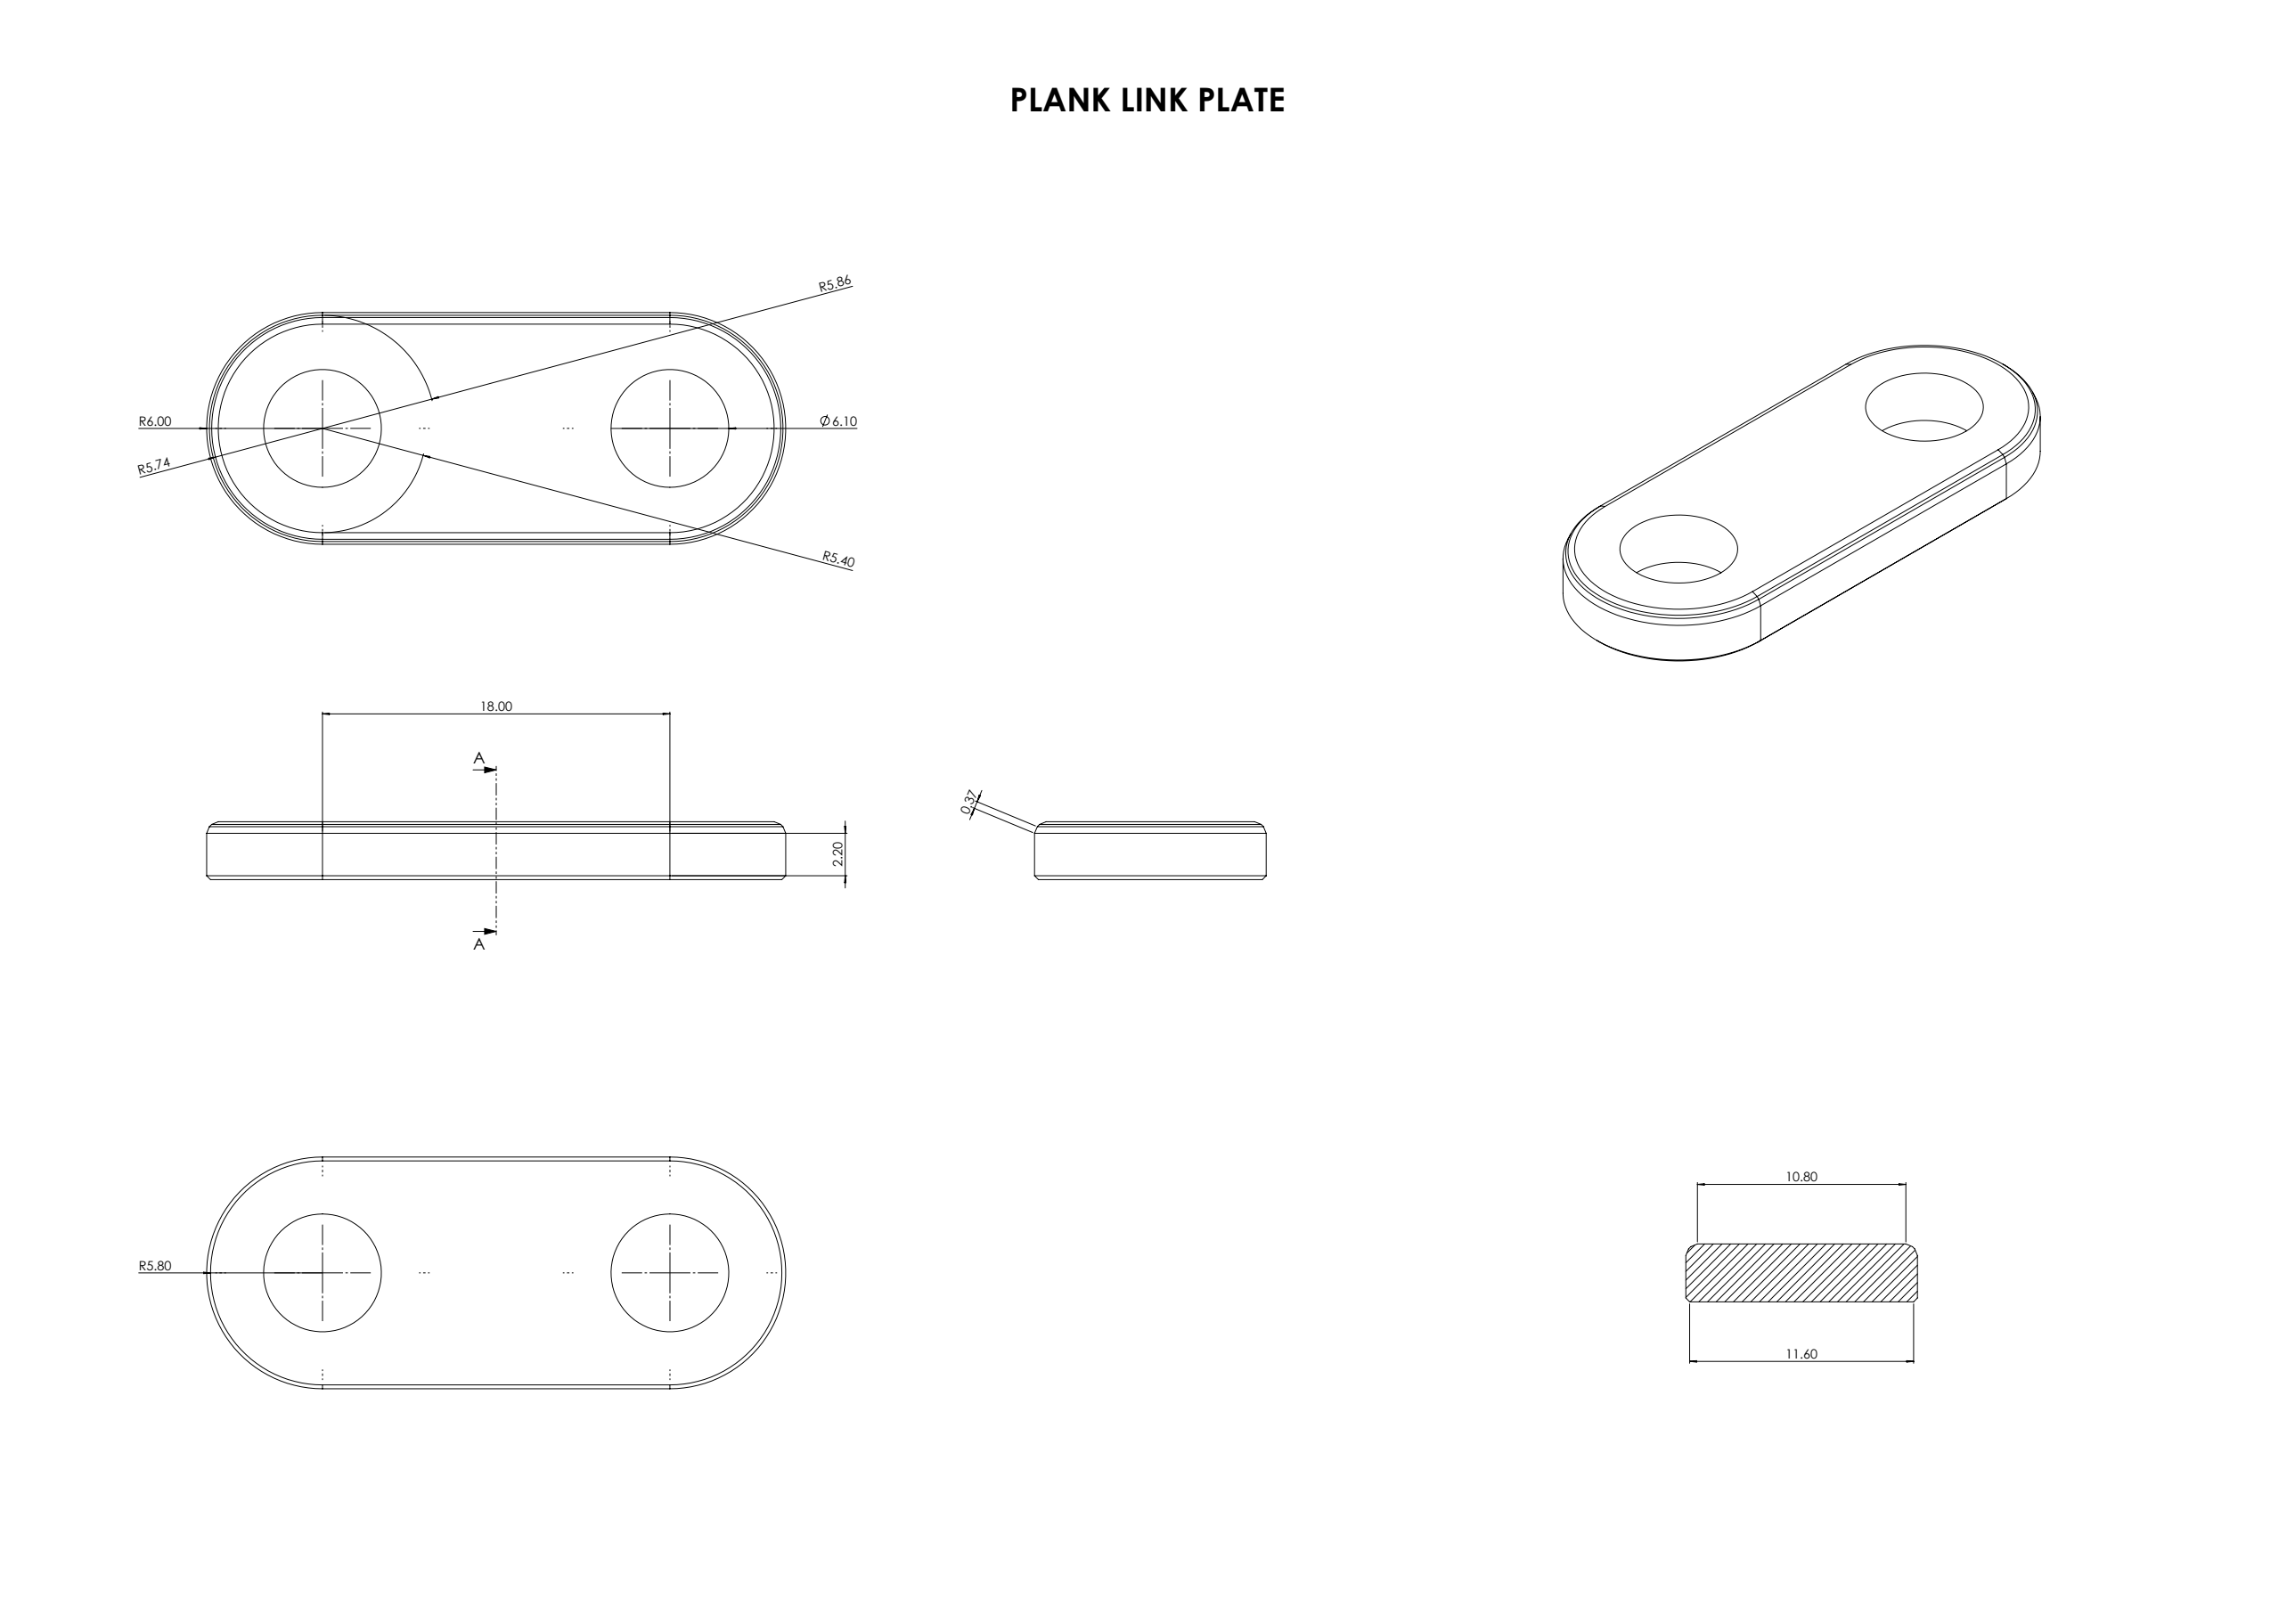
ISO-10303-21;
HEADER;
/* Generated by software containing ST-Developer
 * from STEP Tools, Inc. (www.steptools.com) 
 */

FILE_DESCRIPTION(
/* description */ (''),
/* implementation_level */ '2;1');

FILE_NAME(
/* name */ '09_Plank_Link_Plate.step',
/* time_stamp */ '2026-10-26T03:55:20-07:00',
/* author */ (''),
/* organization */ (''),
/* preprocessor_version */ 'ST-DEVELOPER v20.2',
/* originating_system */ 'Autodesk Translation Framework v15.15.0.0',
/* authorisation */ '');

FILE_SCHEMA (('AUTOMOTIVE_DESIGN { 1 0 10303 214 3 1 1 }'));
ENDSEC;

DATA;
#10=MECHANICAL_DESIGN_GEOMETRIC_PRESENTATION_REPRESENTATION('',(#191),#45236);
#151=SHAPE_REPRESENTATION_RELATIONSHIP('SRR','None',#45330,#171);
#171=ADVANCED_BREP_SHAPE_REPRESENTATION('',(#211),#45232);
#191=STYLED_ITEM('',(#45498),#211);
#211=MANIFOLD_SOLID_BREP('Body1',#16533);
#1051=FACE_BOUND('',#3821,.T.);
#1052=FACE_BOUND('',#3822,.T.);
#1053=FACE_BOUND('',#3835,.T.);
#1054=FACE_BOUND('',#3836,.T.);
#1529=PLANE('',#17991);
#1530=PLANE('',#17995);
#1531=PLANE('',#17996);
#1532=PLANE('',#17999);
#1533=PLANE('',#18002);
#1534=PLANE('',#18005);
#1535=PLANE('',#18011);
#1536=PLANE('',#18012);
#1537=PLANE('',#18015);
#1538=PLANE('',#18020);
#1539=PLANE('',#18023);
#1540=PLANE('',#18027);
#1801=CYLINDRICAL_SURFACE('',#17997,6.);
#1802=CYLINDRICAL_SURFACE('',#18024,3.05);
#1803=CYLINDRICAL_SURFACE('',#18025,3.05);
#1804=CYLINDRICAL_SURFACE('',#18026,6.);
#2728=FACE_OUTER_BOUND('',#3814,.T.);
#2729=FACE_OUTER_BOUND('',#3815,.T.);
#2730=FACE_OUTER_BOUND('',#3816,.T.);
#2731=FACE_OUTER_BOUND('',#3817,.T.);
#2732=FACE_OUTER_BOUND('',#3818,.T.);
#2733=FACE_OUTER_BOUND('',#3819,.T.);
#2734=FACE_OUTER_BOUND('',#3820,.T.);
#2735=FACE_OUTER_BOUND('',#3823,.T.);
#2736=FACE_OUTER_BOUND('',#3824,.T.);
#2737=FACE_OUTER_BOUND('',#3825,.T.);
#2738=FACE_OUTER_BOUND('',#3826,.T.);
#2739=FACE_OUTER_BOUND('',#3827,.T.);
#2740=FACE_OUTER_BOUND('',#3828,.T.);
#2741=FACE_OUTER_BOUND('',#3829,.T.);
#2742=FACE_OUTER_BOUND('',#3830,.T.);
#2743=FACE_OUTER_BOUND('',#3831,.T.);
#2744=FACE_OUTER_BOUND('',#3832,.T.);
#2745=FACE_OUTER_BOUND('',#3833,.T.);
#2746=FACE_OUTER_BOUND('',#3834,.T.);
#2747=FACE_OUTER_BOUND('',#3837,.T.);
#2748=FACE_OUTER_BOUND('',#3838,.T.);
#2749=FACE_OUTER_BOUND('',#3839,.T.);
#2750=FACE_OUTER_BOUND('',#3840,.T.);
#2751=FACE_OUTER_BOUND('',#3841,.T.);
#3814=EDGE_LOOP('',(#15244,#15245,#15246,#15247));
#3815=EDGE_LOOP('',(#15248,#15249,#15250,#15251));
#3816=EDGE_LOOP('',(#15252,#15253,#15254,#15255));
#3817=EDGE_LOOP('',(#15256,#15257,#15258,#15259));
#3818=EDGE_LOOP('',(#15260,#15261,#15262,#15263));
#3819=EDGE_LOOP('',(#15264,#15265,#15266,#15267));
#3820=EDGE_LOOP('',(#15268,#15269,#15270,#15271));
#3821=EDGE_LOOP('',(#15272));
#3822=EDGE_LOOP('',(#15273));
#3823=EDGE_LOOP('',(#15274,#15275,#15276,#15277));
#3824=EDGE_LOOP('',(#15278,#15279,#15280,#15281));
#3825=EDGE_LOOP('',(#15282,#15283,#15284,#15285));
#3826=EDGE_LOOP('',(#15286,#15287,#15288,#15289));
#3827=EDGE_LOOP('',(#15290,#15291,#15292,#15293));
#3828=EDGE_LOOP('',(#15294,#15295,#15296,#15297));
#3829=EDGE_LOOP('',(#15298,#15299,#15300,#15301));
#3830=EDGE_LOOP('',(#15302,#15303,#15304,#15305));
#3831=EDGE_LOOP('',(#15306,#15307,#15308,#15309));
#3832=EDGE_LOOP('',(#15310,#15311,#15312,#15313));
#3833=EDGE_LOOP('',(#15314,#15315,#15316,#15317));
#3834=EDGE_LOOP('',(#15318,#15319,#15320,#15321));
#3835=EDGE_LOOP('',(#15322));
#3836=EDGE_LOOP('',(#15323));
#3837=EDGE_LOOP('',(#15324,#15325,#15326,#15327));
#3838=EDGE_LOOP('',(#15328,#15329,#15330,#15331));
#3839=EDGE_LOOP('',(#15332,#15333,#15334,#15335));
#3840=EDGE_LOOP('',(#15336,#15337,#15338,#15339));
#3841=EDGE_LOOP('',(#15340,#15341,#15342,#15343));
#5125=LINE('',#44904,#6436);
#5126=LINE('',#44908,#6437);
#5127=LINE('',#44913,#6438);
#5128=LINE('',#44914,#6439);
#5129=LINE('',#44915,#6440);
#5130=LINE('',#44919,#6441);
#5131=LINE('',#44923,#6442);
#5132=LINE('',#44924,#6443);
#5133=LINE('',#44927,#6444);
#5134=LINE('',#44929,#6445);
#5135=LINE('',#44930,#6446);
#5136=LINE('',#44933,#6447);
#5137=LINE('',#44942,#6448);
#5138=LINE('',#44944,#6449);
#5139=LINE('',#44945,#6450);
#5140=LINE('',#44948,#6451);
#5141=LINE('',#44953,#6452);
#5142=LINE('',#44954,#6453);
#5143=LINE('',#44955,#6454);
#5144=LINE('',#44961,#6455);
#5145=LINE('',#44964,#6456);
#5146=LINE('',#44967,#6457);
#5147=LINE('',#44968,#6458);
#5148=LINE('',#44971,#6459);
#5149=LINE('',#44973,#6460);
#5150=LINE('',#44974,#6461);
#5151=LINE('',#44977,#6462);
#5152=LINE('',#44982,#6463);
#5153=LINE('',#44983,#6464);
#5154=LINE('',#44984,#6465);
#5155=LINE('',#44989,#6466);
#5156=LINE('',#44997,#6467);
#5157=LINE('',#44999,#6468);
#5158=LINE('',#45001,#6469);
#6436=VECTOR('',#21824,10.);
#6437=VECTOR('',#21827,10.);
#6438=VECTOR('',#21832,10.);
#6439=VECTOR('',#21833,10.);
#6440=VECTOR('',#21834,10.);
#6441=VECTOR('',#21837,10.);
#6442=VECTOR('',#21844,10.);
#6443=VECTOR('',#21845,10.);
#6444=VECTOR('',#21848,10.);
#6445=VECTOR('',#21849,10.);
#6446=VECTOR('',#21850,10.);
#6447=VECTOR('',#21853,10.);
#6448=VECTOR('',#21864,10.);
#6449=VECTOR('',#21865,10.);
#6450=VECTOR('',#21866,10.);
#6451=VECTOR('',#21869,10.);
#6452=VECTOR('',#21874,10.);
#6453=VECTOR('',#21875,10.);
#6454=VECTOR('',#21876,10.);
#6455=VECTOR('',#21885,10.);
#6456=VECTOR('',#21888,10.);
#6457=VECTOR('',#21891,10.);
#6458=VECTOR('',#21892,10.);
#6459=VECTOR('',#21895,10.);
#6460=VECTOR('',#21896,10.);
#6461=VECTOR('',#21897,10.);
#6462=VECTOR('',#21900,10.);
#6463=VECTOR('',#21905,10.);
#6464=VECTOR('',#21906,10.);
#6465=VECTOR('',#21907,10.);
#6466=VECTOR('',#21916,10.);
#6467=VECTOR('',#21927,3.05);
#6468=VECTOR('',#21930,3.05);
#6469=VECTOR('',#21933,10.);
#6922=CIRCLE('',#17989,6.);
#6923=CIRCLE('',#17990,5.8);
#6924=CIRCLE('',#17993,6.);
#6925=CIRCLE('',#17994,5.8);
#6926=CIRCLE('',#17998,6.);
#6927=CIRCLE('',#18000,3.05);
#6928=CIRCLE('',#18001,3.05);
#6929=CIRCLE('',#18004,5.85857864376269);
#6930=CIRCLE('',#18007,5.85857864376269);
#6931=CIRCLE('',#18008,6.);
#6932=CIRCLE('',#18010,5.74142135623731);
#6933=CIRCLE('',#18014,5.4);
#6934=CIRCLE('',#18017,5.74142135623731);
#6935=CIRCLE('',#18018,5.4);
#6936=CIRCLE('',#18021,3.05);
#6937=CIRCLE('',#18022,3.05);
#8395=VERTEX_POINT('',#44902);
#8396=VERTEX_POINT('',#44903);
#8397=VERTEX_POINT('',#44905);
#8398=VERTEX_POINT('',#44907);
#8399=VERTEX_POINT('',#44911);
#8400=VERTEX_POINT('',#44912);
#8401=VERTEX_POINT('',#44917);
#8402=VERTEX_POINT('',#44918);
#8403=VERTEX_POINT('',#44926);
#8404=VERTEX_POINT('',#44928);
#8405=VERTEX_POINT('',#44932);
#8406=VERTEX_POINT('',#44936);
#8407=VERTEX_POINT('',#44938);
#8408=VERTEX_POINT('',#44941);
#8409=VERTEX_POINT('',#44943);
#8410=VERTEX_POINT('',#44947);
#8411=VERTEX_POINT('',#44951);
#8412=VERTEX_POINT('',#44952);
#8413=VERTEX_POINT('',#44960);
#8414=VERTEX_POINT('',#44962);
#8415=VERTEX_POINT('',#44966);
#8416=VERTEX_POINT('',#44970);
#8417=VERTEX_POINT('',#44972);
#8418=VERTEX_POINT('',#44976);
#8419=VERTEX_POINT('',#44980);
#8420=VERTEX_POINT('',#44981);
#8421=VERTEX_POINT('',#44991);
#8422=VERTEX_POINT('',#44993);
#10685=EDGE_CURVE('',#8395,#8396,#5125,.T.);
#10686=EDGE_CURVE('',#8396,#8397,#6922,.T.);
#10687=EDGE_CURVE('',#8397,#8398,#5126,.T.);
#10688=EDGE_CURVE('',#8398,#8395,#6923,.T.);
#10689=EDGE_CURVE('',#8399,#8400,#5127,.T.);
#10690=EDGE_CURVE('',#8400,#8396,#5128,.T.);
#10691=EDGE_CURVE('',#8395,#8399,#5129,.T.);
#10692=EDGE_CURVE('',#8401,#8402,#5130,.T.);
#10693=EDGE_CURVE('',#8402,#8400,#6924,.T.);
#10694=EDGE_CURVE('',#8399,#8401,#6925,.T.);
#10695=EDGE_CURVE('',#8397,#8402,#5131,.T.);
#10696=EDGE_CURVE('',#8401,#8398,#5132,.T.);
#10697=EDGE_CURVE('',#8397,#8403,#5133,.T.);
#10698=EDGE_CURVE('',#8404,#8403,#5134,.T.);
#10699=EDGE_CURVE('',#8402,#8404,#5135,.T.);
#10700=EDGE_CURVE('',#8396,#8405,#5136,.T.);
#10701=EDGE_CURVE('',#8403,#8405,#6926,.T.);
#10702=EDGE_CURVE('',#8406,#8406,#6927,.T.);
#10703=EDGE_CURVE('',#8407,#8407,#6928,.T.);
#10704=EDGE_CURVE('',#8403,#8408,#5137,.T.);
#10705=EDGE_CURVE('',#8408,#8409,#5138,.T.);
#10706=EDGE_CURVE('',#8409,#8404,#5139,.T.);
#10707=EDGE_CURVE('',#8405,#8410,#5140,.T.);
#10708=EDGE_CURVE('',#8410,#8408,#6929,.T.);
#10709=EDGE_CURVE('',#8411,#8412,#5141,.T.);
#10710=EDGE_CURVE('',#8412,#8410,#5142,.T.);
#10711=EDGE_CURVE('',#8405,#8411,#5143,.T.);
#10712=EDGE_CURVE('',#8409,#8412,#6930,.T.);
#10713=EDGE_CURVE('',#8411,#8404,#6931,.T.);
#10714=EDGE_CURVE('',#8413,#8409,#5144,.T.);
#10715=EDGE_CURVE('',#8414,#8413,#6932,.T.);
#10716=EDGE_CURVE('',#8412,#8414,#5145,.T.);
#10717=EDGE_CURVE('',#8408,#8415,#5146,.T.);
#10718=EDGE_CURVE('',#8413,#8415,#5147,.T.);
#10719=EDGE_CURVE('',#8416,#8413,#5148,.T.);
#10720=EDGE_CURVE('',#8415,#8417,#5149,.T.);
#10721=EDGE_CURVE('',#8417,#8416,#5150,.T.);
#10722=EDGE_CURVE('',#8418,#8414,#5151,.T.);
#10723=EDGE_CURVE('',#8416,#8418,#6933,.T.);
#10724=EDGE_CURVE('',#8419,#8420,#5152,.T.);
#10725=EDGE_CURVE('',#8420,#8414,#5153,.T.);
#10726=EDGE_CURVE('',#8418,#8419,#5154,.T.);
#10727=EDGE_CURVE('',#8415,#8420,#6934,.T.);
#10728=EDGE_CURVE('',#8419,#8417,#6935,.T.);
#10729=EDGE_CURVE('',#8410,#8420,#5155,.T.);
#10730=EDGE_CURVE('',#8421,#8421,#6936,.T.);
#10731=EDGE_CURVE('',#8422,#8422,#6937,.T.);
#10732=EDGE_CURVE('',#8407,#8421,#5156,.T.);
#10733=EDGE_CURVE('',#8406,#8422,#5157,.T.);
#10734=EDGE_CURVE('',#8400,#8411,#5158,.T.);
#15244=ORIENTED_EDGE('',*,*,#10685,.T.);
#15245=ORIENTED_EDGE('',*,*,#10686,.T.);
#15246=ORIENTED_EDGE('',*,*,#10687,.T.);
#15247=ORIENTED_EDGE('',*,*,#10688,.T.);
#15248=ORIENTED_EDGE('',*,*,#10689,.T.);
#15249=ORIENTED_EDGE('',*,*,#10690,.T.);
#15250=ORIENTED_EDGE('',*,*,#10685,.F.);
#15251=ORIENTED_EDGE('',*,*,#10691,.T.);
#15252=ORIENTED_EDGE('',*,*,#10692,.T.);
#15253=ORIENTED_EDGE('',*,*,#10693,.T.);
#15254=ORIENTED_EDGE('',*,*,#10689,.F.);
#15255=ORIENTED_EDGE('',*,*,#10694,.T.);
#15256=ORIENTED_EDGE('',*,*,#10687,.F.);
#15257=ORIENTED_EDGE('',*,*,#10695,.T.);
#15258=ORIENTED_EDGE('',*,*,#10692,.F.);
#15259=ORIENTED_EDGE('',*,*,#10696,.T.);
#15260=ORIENTED_EDGE('',*,*,#10695,.F.);
#15261=ORIENTED_EDGE('',*,*,#10697,.T.);
#15262=ORIENTED_EDGE('',*,*,#10698,.F.);
#15263=ORIENTED_EDGE('',*,*,#10699,.F.);
#15264=ORIENTED_EDGE('',*,*,#10686,.F.);
#15265=ORIENTED_EDGE('',*,*,#10700,.T.);
#15266=ORIENTED_EDGE('',*,*,#10701,.F.);
#15267=ORIENTED_EDGE('',*,*,#10697,.F.);
#15268=ORIENTED_EDGE('',*,*,#10688,.F.);
#15269=ORIENTED_EDGE('',*,*,#10696,.F.);
#15270=ORIENTED_EDGE('',*,*,#10694,.F.);
#15271=ORIENTED_EDGE('',*,*,#10691,.F.);
#15272=ORIENTED_EDGE('',*,*,#10702,.T.);
#15273=ORIENTED_EDGE('',*,*,#10703,.T.);
#15274=ORIENTED_EDGE('',*,*,#10704,.T.);
#15275=ORIENTED_EDGE('',*,*,#10705,.T.);
#15276=ORIENTED_EDGE('',*,*,#10706,.T.);
#15277=ORIENTED_EDGE('',*,*,#10698,.T.);
#15278=ORIENTED_EDGE('',*,*,#10707,.T.);
#15279=ORIENTED_EDGE('',*,*,#10708,.T.);
#15280=ORIENTED_EDGE('',*,*,#10704,.F.);
#15281=ORIENTED_EDGE('',*,*,#10701,.T.);
#15282=ORIENTED_EDGE('',*,*,#10709,.T.);
#15283=ORIENTED_EDGE('',*,*,#10710,.T.);
#15284=ORIENTED_EDGE('',*,*,#10707,.F.);
#15285=ORIENTED_EDGE('',*,*,#10711,.T.);
#15286=ORIENTED_EDGE('',*,*,#10706,.F.);
#15287=ORIENTED_EDGE('',*,*,#10712,.T.);
#15288=ORIENTED_EDGE('',*,*,#10709,.F.);
#15289=ORIENTED_EDGE('',*,*,#10713,.T.);
#15290=ORIENTED_EDGE('',*,*,#10712,.F.);
#15291=ORIENTED_EDGE('',*,*,#10714,.F.);
#15292=ORIENTED_EDGE('',*,*,#10715,.F.);
#15293=ORIENTED_EDGE('',*,*,#10716,.F.);
#15294=ORIENTED_EDGE('',*,*,#10705,.F.);
#15295=ORIENTED_EDGE('',*,*,#10717,.T.);
#15296=ORIENTED_EDGE('',*,*,#10718,.F.);
#15297=ORIENTED_EDGE('',*,*,#10714,.T.);
#15298=ORIENTED_EDGE('',*,*,#10719,.T.);
#15299=ORIENTED_EDGE('',*,*,#10718,.T.);
#15300=ORIENTED_EDGE('',*,*,#10720,.T.);
#15301=ORIENTED_EDGE('',*,*,#10721,.T.);
#15302=ORIENTED_EDGE('',*,*,#10722,.T.);
#15303=ORIENTED_EDGE('',*,*,#10715,.T.);
#15304=ORIENTED_EDGE('',*,*,#10719,.F.);
#15305=ORIENTED_EDGE('',*,*,#10723,.T.);
#15306=ORIENTED_EDGE('',*,*,#10724,.T.);
#15307=ORIENTED_EDGE('',*,*,#10725,.T.);
#15308=ORIENTED_EDGE('',*,*,#10722,.F.);
#15309=ORIENTED_EDGE('',*,*,#10726,.T.);
#15310=ORIENTED_EDGE('',*,*,#10720,.F.);
#15311=ORIENTED_EDGE('',*,*,#10727,.T.);
#15312=ORIENTED_EDGE('',*,*,#10724,.F.);
#15313=ORIENTED_EDGE('',*,*,#10728,.T.);
#15314=ORIENTED_EDGE('',*,*,#10708,.F.);
#15315=ORIENTED_EDGE('',*,*,#10729,.T.);
#15316=ORIENTED_EDGE('',*,*,#10727,.F.);
#15317=ORIENTED_EDGE('',*,*,#10717,.F.);
#15318=ORIENTED_EDGE('',*,*,#10721,.F.);
#15319=ORIENTED_EDGE('',*,*,#10728,.F.);
#15320=ORIENTED_EDGE('',*,*,#10726,.F.);
#15321=ORIENTED_EDGE('',*,*,#10723,.F.);
#15322=ORIENTED_EDGE('',*,*,#10730,.T.);
#15323=ORIENTED_EDGE('',*,*,#10731,.T.);
#15324=ORIENTED_EDGE('',*,*,#10710,.F.);
#15325=ORIENTED_EDGE('',*,*,#10716,.T.);
#15326=ORIENTED_EDGE('',*,*,#10725,.F.);
#15327=ORIENTED_EDGE('',*,*,#10729,.F.);
#15328=ORIENTED_EDGE('',*,*,#10703,.F.);
#15329=ORIENTED_EDGE('',*,*,#10732,.T.);
#15330=ORIENTED_EDGE('',*,*,#10730,.F.);
#15331=ORIENTED_EDGE('',*,*,#10732,.F.);
#15332=ORIENTED_EDGE('',*,*,#10702,.F.);
#15333=ORIENTED_EDGE('',*,*,#10733,.T.);
#15334=ORIENTED_EDGE('',*,*,#10731,.F.);
#15335=ORIENTED_EDGE('',*,*,#10733,.F.);
#15336=ORIENTED_EDGE('',*,*,#10693,.F.);
#15337=ORIENTED_EDGE('',*,*,#10699,.T.);
#15338=ORIENTED_EDGE('',*,*,#10713,.F.);
#15339=ORIENTED_EDGE('',*,*,#10734,.F.);
#15340=ORIENTED_EDGE('',*,*,#10690,.F.);
#15341=ORIENTED_EDGE('',*,*,#10734,.T.);
#15342=ORIENTED_EDGE('',*,*,#10711,.F.);
#15343=ORIENTED_EDGE('',*,*,#10700,.F.);
#15530=CONICAL_SURFACE('',#17988,5.9,0.785398163397448);
#15531=CONICAL_SURFACE('',#17992,5.9,0.785398163397448);
#15532=CONICAL_SURFACE('',#18003,5.92928932188135,0.392699081698723);
#15533=CONICAL_SURFACE('',#18006,5.92928932188134,0.392699081698725);
#15534=CONICAL_SURFACE('',#18009,5.8,0.785398163397448);
#15535=CONICAL_SURFACE('',#18013,5.57071067811865,1.17809724509617);
#15536=CONICAL_SURFACE('',#18016,5.57071067811865,1.17809724509617);
#15537=CONICAL_SURFACE('',#18019,5.8,0.785398163397448);
#16456=ADVANCED_FACE('',(#2728),#15530,.T.);
#16457=ADVANCED_FACE('',(#2729),#1529,.T.);
#16458=ADVANCED_FACE('',(#2730),#15531,.T.);
#16459=ADVANCED_FACE('',(#2731),#1530,.T.);
#16460=ADVANCED_FACE('',(#2732),#1531,.T.);
#16461=ADVANCED_FACE('',(#2733),#1801,.T.);
#16462=ADVANCED_FACE('',(#2734,#1051,#1052),#1532,.F.);
#16463=ADVANCED_FACE('',(#2735),#1533,.T.);
#16464=ADVANCED_FACE('',(#2736),#15532,.T.);
#16465=ADVANCED_FACE('',(#2737),#1534,.T.);
#16466=ADVANCED_FACE('',(#2738),#15533,.T.);
#16467=ADVANCED_FACE('',(#2739),#15534,.T.);
#16468=ADVANCED_FACE('',(#2740),#1535,.T.);
#16469=ADVANCED_FACE('',(#2741),#1536,.T.);
#16470=ADVANCED_FACE('',(#2742),#15535,.T.);
#16471=ADVANCED_FACE('',(#2743),#1537,.T.);
#16472=ADVANCED_FACE('',(#2744),#15536,.T.);
#16473=ADVANCED_FACE('',(#2745),#15537,.T.);
#16474=ADVANCED_FACE('',(#2746,#1053,#1054),#1538,.T.);
#16475=ADVANCED_FACE('',(#2747),#1539,.T.);
#16476=ADVANCED_FACE('',(#2748),#1802,.F.);
#16477=ADVANCED_FACE('',(#2749),#1803,.F.);
#16478=ADVANCED_FACE('',(#2750),#1804,.T.);
#16479=ADVANCED_FACE('',(#2751),#1540,.T.);
#16533=CLOSED_SHELL('',(#16456,#16457,#16458,#16459,#16460,#16461,#16462,
#16463,#16464,#16465,#16466,#16467,#16468,#16469,#16470,#16471,#16472,#16473,
#16474,#16475,#16476,#16477,#16478,#16479));
#17987=AXIS2_PLACEMENT_3D('',#44900,#21820,#21821);
#17988=AXIS2_PLACEMENT_3D('',#44901,#21822,#21823);
#17989=AXIS2_PLACEMENT_3D('',#44906,#21825,#21826);
#17990=AXIS2_PLACEMENT_3D('',#44909,#21828,#21829);
#17991=AXIS2_PLACEMENT_3D('',#44910,#21830,#21831);
#17992=AXIS2_PLACEMENT_3D('',#44916,#21835,#21836);
#17993=AXIS2_PLACEMENT_3D('',#44920,#21838,#21839);
#17994=AXIS2_PLACEMENT_3D('',#44921,#21840,#21841);
#17995=AXIS2_PLACEMENT_3D('',#44922,#21842,#21843);
#17996=AXIS2_PLACEMENT_3D('',#44925,#21846,#21847);
#17997=AXIS2_PLACEMENT_3D('',#44931,#21851,#21852);
#17998=AXIS2_PLACEMENT_3D('',#44934,#21854,#21855);
#17999=AXIS2_PLACEMENT_3D('',#44935,#21856,#21857);
#18000=AXIS2_PLACEMENT_3D('',#44937,#21858,#21859);
#18001=AXIS2_PLACEMENT_3D('',#44939,#21860,#21861);
#18002=AXIS2_PLACEMENT_3D('',#44940,#21862,#21863);
#18003=AXIS2_PLACEMENT_3D('',#44946,#21867,#21868);
#18004=AXIS2_PLACEMENT_3D('',#44949,#21870,#21871);
#18005=AXIS2_PLACEMENT_3D('',#44950,#21872,#21873);
#18006=AXIS2_PLACEMENT_3D('',#44956,#21877,#21878);
#18007=AXIS2_PLACEMENT_3D('',#44957,#21879,#21880);
#18008=AXIS2_PLACEMENT_3D('',#44958,#21881,#21882);
#18009=AXIS2_PLACEMENT_3D('',#44959,#21883,#21884);
#18010=AXIS2_PLACEMENT_3D('',#44963,#21886,#21887);
#18011=AXIS2_PLACEMENT_3D('',#44965,#21889,#21890);
#18012=AXIS2_PLACEMENT_3D('',#44969,#21893,#21894);
#18013=AXIS2_PLACEMENT_3D('',#44975,#21898,#21899);
#18014=AXIS2_PLACEMENT_3D('',#44978,#21901,#21902);
#18015=AXIS2_PLACEMENT_3D('',#44979,#21903,#21904);
#18016=AXIS2_PLACEMENT_3D('',#44985,#21908,#21909);
#18017=AXIS2_PLACEMENT_3D('',#44986,#21910,#21911);
#18018=AXIS2_PLACEMENT_3D('',#44987,#21912,#21913);
#18019=AXIS2_PLACEMENT_3D('',#44988,#21914,#21915);
#18020=AXIS2_PLACEMENT_3D('',#44990,#21917,#21918);
#18021=AXIS2_PLACEMENT_3D('',#44992,#21919,#21920);
#18022=AXIS2_PLACEMENT_3D('',#44994,#21921,#21922);
#18023=AXIS2_PLACEMENT_3D('',#44995,#21923,#21924);
#18024=AXIS2_PLACEMENT_3D('',#44996,#21925,#21926);
#18025=AXIS2_PLACEMENT_3D('',#44998,#21928,#21929);
#18026=AXIS2_PLACEMENT_3D('',#45000,#21931,#21932);
#18027=AXIS2_PLACEMENT_3D('',#45002,#21934,#21935);
#21820=DIRECTION('axis',(0.,0.,1.));
#21821=DIRECTION('refdir',(1.,0.,0.));
#21822=DIRECTION('center_axis',(0.,1.,0.));
#21823=DIRECTION('ref_axis',(1.,0.,0.));
#21824=DIRECTION('',(-0.707106781186548,0.707106781186548,-8.65956056235495E-17));
#21825=DIRECTION('center_axis',(0.,-1.,0.));
#21826=DIRECTION('ref_axis',(1.,0.,0.));
#21827=DIRECTION('',(-0.707106781186548,-0.707106781186548,0.));
#21828=DIRECTION('center_axis',(0.,1.,0.));
#21829=DIRECTION('ref_axis',(1.,0.,0.));
#21830=DIRECTION('center_axis',(-0.707106781186548,-0.707106781186548,0.));
#21831=DIRECTION('ref_axis',(0.,0.,1.));
#21832=DIRECTION('',(-0.707106781186548,0.707106781186548,0.));
#21833=DIRECTION('',(0.,0.,-1.));
#21834=DIRECTION('',(0.,0.,1.));
#21835=DIRECTION('center_axis',(0.,1.,0.));
#21836=DIRECTION('ref_axis',(-1.,0.,0.));
#21837=DIRECTION('',(0.707106781186548,0.707106781186548,0.));
#21838=DIRECTION('center_axis',(0.,-1.,0.));
#21839=DIRECTION('ref_axis',(-1.,0.,0.));
#21840=DIRECTION('center_axis',(0.,1.,0.));
#21841=DIRECTION('ref_axis',(-1.,0.,0.));
#21842=DIRECTION('center_axis',(0.707106781186548,-0.707106781186548,0.));
#21843=DIRECTION('ref_axis',(0.,0.,-1.));
#21844=DIRECTION('',(0.,0.,1.));
#21845=DIRECTION('',(0.,0.,-1.));
#21846=DIRECTION('center_axis',(1.,0.,0.));
#21847=DIRECTION('ref_axis',(0.,0.,-1.));
#21848=DIRECTION('',(0.,1.,0.));
#21849=DIRECTION('',(0.,0.,-1.));
#21850=DIRECTION('',(0.,1.,0.));
#21851=DIRECTION('center_axis',(0.,1.,0.));
#21852=DIRECTION('ref_axis',(1.,0.,0.));
#21853=DIRECTION('',(0.,1.,0.));
#21854=DIRECTION('center_axis',(0.,1.,0.));
#21855=DIRECTION('ref_axis',(1.,0.,0.));
#21856=DIRECTION('center_axis',(0.,1.,0.));
#21857=DIRECTION('ref_axis',(1.,0.,0.));
#21858=DIRECTION('center_axis',(0.,1.,0.));
#21859=DIRECTION('ref_axis',(1.,0.,0.));
#21860=DIRECTION('center_axis',(0.,1.,0.));
#21861=DIRECTION('ref_axis',(1.,0.,0.));
#21862=DIRECTION('center_axis',(0.923879532511287,0.382683432365089,0.));
#21863=DIRECTION('ref_axis',(0.,0.,-1.));
#21864=DIRECTION('',(-0.382683432365089,0.923879532511287,0.));
#21865=DIRECTION('',(0.,0.,1.));
#21866=DIRECTION('',(0.382683432365089,-0.923879532511287,0.));
#21867=DIRECTION('center_axis',(0.,-1.,-1.0507089630694E-15));
#21868=DIRECTION('ref_axis',(1.,0.,-3.02510519985914E-17));
#21869=DIRECTION('',(0.382683432365089,0.923879532511287,4.68652040532631E-17));
#21870=DIRECTION('center_axis',(0.,-1.,0.));
#21871=DIRECTION('ref_axis',(1.,0.,-6.12323399573676E-17));
#21872=DIRECTION('center_axis',(-0.923879532511287,0.382683432365089,0.));
#21873=DIRECTION('ref_axis',(0.,0.,1.));
#21874=DIRECTION('',(0.382683432365089,0.923879532511287,0.));
#21875=DIRECTION('',(0.,0.,-1.));
#21876=DIRECTION('',(0.,0.,1.));
#21877=DIRECTION('center_axis',(0.,-1.,0.));
#21878=DIRECTION('ref_axis',(-1.,0.,0.));
#21879=DIRECTION('center_axis',(0.,-1.,0.));
#21880=DIRECTION('ref_axis',(-1.,0.,0.));
#21881=DIRECTION('center_axis',(0.,1.,0.));
#21882=DIRECTION('ref_axis',(-1.,0.,0.));
#21883=DIRECTION('center_axis',(0.,-1.,0.));
#21884=DIRECTION('ref_axis',(-1.,0.,0.));
#21885=DIRECTION('',(0.707106781186548,-0.707106781186548,0.));
#21886=DIRECTION('center_axis',(0.,1.,0.));
#21887=DIRECTION('ref_axis',(-1.,0.,0.));
#21888=DIRECTION('',(0.707106781186548,0.707106781186548,0.));
#21889=DIRECTION('center_axis',(0.707106781186548,0.707106781186548,0.));
#21890=DIRECTION('ref_axis',(0.,0.,-1.));
#21891=DIRECTION('',(-0.707106781186548,0.707106781186548,0.));
#21892=DIRECTION('',(0.,0.,-1.));
#21893=DIRECTION('center_axis',(0.382683432365093,0.923879532511286,0.));
#21894=DIRECTION('ref_axis',(0.,0.,1.));
#21895=DIRECTION('',(0.923879532511286,-0.382683432365093,0.));
#21896=DIRECTION('',(-0.923879532511286,0.382683432365093,0.));
#21897=DIRECTION('',(0.,0.,1.));
#21898=DIRECTION('center_axis',(0.,-1.,0.));
#21899=DIRECTION('ref_axis',(-1.,0.,0.));
#21900=DIRECTION('',(-0.923879532511286,-0.38268343236509,-6.00848371219648E-15));
#21901=DIRECTION('center_axis',(0.,-1.,0.));
#21902=DIRECTION('ref_axis',(-1.,0.,0.));
#21903=DIRECTION('center_axis',(-0.382683432365093,0.923879532511286,0.));
#21904=DIRECTION('ref_axis',(0.,0.,1.));
#21905=DIRECTION('',(-0.923879532511286,-0.382683432365093,1.10160925113079E-15));
#21906=DIRECTION('',(0.,0.,1.));
#21907=DIRECTION('',(0.,0.,-1.));
#21908=DIRECTION('center_axis',(0.,-1.,2.48590929741676E-15));
#21909=DIRECTION('ref_axis',(1.,0.,-3.15543818946224E-17));
#21910=DIRECTION('center_axis',(0.,1.,0.));
#21911=DIRECTION('ref_axis',(1.,0.,-6.12323399573677E-17));
#21912=DIRECTION('center_axis',(0.,-1.,0.));
#21913=DIRECTION('ref_axis',(1.,0.,0.));
#21914=DIRECTION('center_axis',(0.,-1.,0.));
#21915=DIRECTION('ref_axis',(1.,0.,0.));
#21916=DIRECTION('',(0.707106781186548,0.707106781186548,8.65956056235493E-17));
#21917=DIRECTION('center_axis',(0.,1.,0.));
#21918=DIRECTION('ref_axis',(1.,0.,0.));
#21919=DIRECTION('center_axis',(0.,-1.,0.));
#21920=DIRECTION('ref_axis',(1.,0.,0.));
#21921=DIRECTION('center_axis',(0.,-1.,0.));
#21922=DIRECTION('ref_axis',(1.,0.,0.));
#21923=DIRECTION('center_axis',(-0.707106781186548,0.707106781186548,0.));
#21924=DIRECTION('ref_axis',(0.,0.,1.));
#21925=DIRECTION('center_axis',(0.,1.,0.));
#21926=DIRECTION('ref_axis',(1.,0.,0.));
#21927=DIRECTION('',(0.,1.,0.));
#21928=DIRECTION('center_axis',(0.,1.,0.));
#21929=DIRECTION('ref_axis',(1.,0.,0.));
#21930=DIRECTION('',(0.,1.,0.));
#21931=DIRECTION('center_axis',(0.,1.,0.));
#21932=DIRECTION('ref_axis',(-1.,0.,0.));
#21933=DIRECTION('',(0.,1.,0.));
#21934=DIRECTION('center_axis',(-1.,0.,0.));
#21935=DIRECTION('ref_axis',(0.,0.,1.));
#44900=CARTESIAN_POINT('',(0.,0.,0.));
#44901=CARTESIAN_POINT('Origin',(0.,5.1,0.));
#44902=CARTESIAN_POINT('',(-5.8,5.,-7.10295143505465E-16));
#44903=CARTESIAN_POINT('',(-6.,5.2,-7.34788079488412E-16));
#44904=CARTESIAN_POINT('',(-5.8,5.,-7.10295143505465E-16));
#44905=CARTESIAN_POINT('',(6.,5.2,0.));
#44906=CARTESIAN_POINT('Origin',(0.,5.2,0.));
#44907=CARTESIAN_POINT('',(5.8,5.,0.));
#44908=CARTESIAN_POINT('',(6.,5.2,0.));
#44909=CARTESIAN_POINT('Origin',(0.,5.,0.));
#44910=CARTESIAN_POINT('Origin',(-5.9,5.1,4.5));
#44911=CARTESIAN_POINT('',(-5.8,5.,18.));
#44912=CARTESIAN_POINT('',(-6.,5.2,18.));
#44913=CARTESIAN_POINT('',(-5.8,5.,18.));
#44914=CARTESIAN_POINT('',(-6.,5.2,4.5));
#44915=CARTESIAN_POINT('',(-5.8,5.,4.5));
#44916=CARTESIAN_POINT('Origin',(0.,5.1,18.));
#44917=CARTESIAN_POINT('',(5.8,5.,18.));
#44918=CARTESIAN_POINT('',(6.,5.2,18.));
#44919=CARTESIAN_POINT('',(5.8,5.,18.));
#44920=CARTESIAN_POINT('Origin',(0.,5.2,18.));
#44921=CARTESIAN_POINT('Origin',(0.,5.,18.));
#44922=CARTESIAN_POINT('Origin',(5.9,5.1,13.5));
#44923=CARTESIAN_POINT('',(6.,5.2,13.5));
#44924=CARTESIAN_POINT('',(5.8,5.,13.5));
#44925=CARTESIAN_POINT('Origin',(6.,5.,18.));
#44926=CARTESIAN_POINT('',(6.,7.4,0.));
#44927=CARTESIAN_POINT('',(6.,5.,0.));
#44928=CARTESIAN_POINT('',(6.,7.4,18.));
#44929=CARTESIAN_POINT('',(6.,7.4,15.75));
#44930=CARTESIAN_POINT('',(6.,5.,18.));
#44931=CARTESIAN_POINT('Origin',(0.,5.,0.));
#44932=CARTESIAN_POINT('',(-6.,7.4,-7.34788079488412E-16));
#44933=CARTESIAN_POINT('',(-6.,5.,-7.34788079488412E-16));
#44934=CARTESIAN_POINT('Origin',(0.,7.4,0.));
#44935=CARTESIAN_POINT('Origin',(0.,5.,9.));
#44936=CARTESIAN_POINT('',(-3.05,5.,18.));
#44937=CARTESIAN_POINT('Origin',(0.,5.,18.));
#44938=CARTESIAN_POINT('',(-3.05,5.,3.73517273739943E-16));
#44939=CARTESIAN_POINT('Origin',(0.,5.,0.));
#44940=CARTESIAN_POINT('Origin',(5.92928932188135,7.57071067811865,15.75));
#44941=CARTESIAN_POINT('',(5.85857864376269,7.74142135623731,0.));
#44942=CARTESIAN_POINT('',(6.,7.4,0.));
#44943=CARTESIAN_POINT('',(5.85857864376269,7.74142135623731,18.));
#44944=CARTESIAN_POINT('',(5.85857864376269,7.74142135623731,15.75));
#44945=CARTESIAN_POINT('',(5.85857864376269,7.74142135623731,18.));
#44946=CARTESIAN_POINT('Origin',(0.,7.57071067811865,1.79367239590926E-16));
#44947=CARTESIAN_POINT('',(-5.85857864376269,7.74142135623731,-7.17468958363702E-16));
#44948=CARTESIAN_POINT('',(-6.,7.4,-7.34788079488412E-16));
#44949=CARTESIAN_POINT('Origin',(0.,7.74142135623731,3.58734479181851E-16));
#44950=CARTESIAN_POINT('Origin',(-5.92928932188135,7.57071067811865,2.25));
#44951=CARTESIAN_POINT('',(-6.,7.4,18.));
#44952=CARTESIAN_POINT('',(-5.85857864376269,7.74142135623731,18.));
#44953=CARTESIAN_POINT('',(-6.,7.4,18.));
#44954=CARTESIAN_POINT('',(-5.85857864376269,7.74142135623731,2.25));
#44955=CARTESIAN_POINT('',(-6.,7.4,2.25));
#44956=CARTESIAN_POINT('Origin',(0.,7.57071067811865,18.));
#44957=CARTESIAN_POINT('Origin',(0.,7.74142135623731,18.));
#44958=CARTESIAN_POINT('Origin',(0.,7.4,18.));
#44959=CARTESIAN_POINT('Origin',(0.,7.8,18.));
#44960=CARTESIAN_POINT('',(5.74142135623731,7.85857864376269,18.));
#44961=CARTESIAN_POINT('',(5.6,8.,18.));
#44962=CARTESIAN_POINT('',(-5.74142135623731,7.85857864376269,18.));
#44963=CARTESIAN_POINT('Origin',(0.,7.85857864376269,18.));
#44964=CARTESIAN_POINT('',(-6.,7.6,18.));
#44965=CARTESIAN_POINT('Origin',(5.8,7.8,13.5));
#44966=CARTESIAN_POINT('',(5.74142135623731,7.85857864376269,0.));
#44967=CARTESIAN_POINT('',(6.,7.6,0.));
#44968=CARTESIAN_POINT('',(5.74142135623731,7.85857864376269,11.25));
#44969=CARTESIAN_POINT('Origin',(5.57071067811865,7.92928932188135,11.25));
#44970=CARTESIAN_POINT('',(5.4,8.,18.));
#44971=CARTESIAN_POINT('',(5.4,8.,18.));
#44972=CARTESIAN_POINT('',(5.4,8.,0.));
#44973=CARTESIAN_POINT('',(5.74142135623731,7.85857864376269,0.));
#44974=CARTESIAN_POINT('',(5.4,8.,11.25));
#44975=CARTESIAN_POINT('Origin',(0.,7.92928932188135,18.));
#44976=CARTESIAN_POINT('',(-5.4,8.,18.));
#44977=CARTESIAN_POINT('',(-5.4,8.,18.));
#44978=CARTESIAN_POINT('Origin',(0.,8.,18.));
#44979=CARTESIAN_POINT('Origin',(-5.57071067811865,7.92928932188135,6.75));
#44980=CARTESIAN_POINT('',(-5.4,8.,-1.11022302462516E-15));
#44981=CARTESIAN_POINT('',(-5.74142135623731,7.85857864376269,-7.03121328647228E-16));
#44982=CARTESIAN_POINT('',(-5.4,8.,-1.11022302462516E-15));
#44983=CARTESIAN_POINT('',(-5.74142135623731,7.85857864376269,6.75));
#44984=CARTESIAN_POINT('',(-5.4,8.,6.75));
#44985=CARTESIAN_POINT('Origin',(0.,7.92928932188135,1.75780332161807E-16));
#44986=CARTESIAN_POINT('Origin',(0.,7.85857864376269,3.51560664323614E-16));
#44987=CARTESIAN_POINT('Origin',(0.,8.,0.));
#44988=CARTESIAN_POINT('Origin',(0.,7.8,0.));
#44989=CARTESIAN_POINT('',(-6.,7.6,-7.34788079488412E-16));
#44990=CARTESIAN_POINT('Origin',(0.,8.,9.));
#44991=CARTESIAN_POINT('',(-3.05,8.,-3.73517273739943E-16));
#44992=CARTESIAN_POINT('Origin',(0.,8.,0.));
#44993=CARTESIAN_POINT('',(-3.05,8.,18.));
#44994=CARTESIAN_POINT('Origin',(0.,8.,18.));
#44995=CARTESIAN_POINT('Origin',(-5.8,7.8,4.5));
#44996=CARTESIAN_POINT('Origin',(0.,4.9,0.));
#44997=CARTESIAN_POINT('',(-3.05,4.9,3.73517273739943E-16));
#44998=CARTESIAN_POINT('Origin',(0.,4.9,18.));
#44999=CARTESIAN_POINT('',(-3.05,4.9,18.));
#45000=CARTESIAN_POINT('Origin',(0.,5.,18.));
#45001=CARTESIAN_POINT('',(-6.,5.,18.));
#45002=CARTESIAN_POINT('Origin',(-6.,5.,0.));
#45210=UNCERTAINTY_MEASURE_WITH_UNIT(LENGTH_MEASURE(0.01),#45237,
'DISTANCE_ACCURACY_VALUE',
'Maximum model space distance between geometric entities at asserted c
onnectivities');
#45214=UNCERTAINTY_MEASURE_WITH_UNIT(LENGTH_MEASURE(0.01),#45237,
'DISTANCE_ACCURACY_VALUE',
'Maximum model space distance between geometric entities at asserted c
onnectivities');
#45232=(
GEOMETRIC_REPRESENTATION_CONTEXT(3)
GLOBAL_UNCERTAINTY_ASSIGNED_CONTEXT((#45210))
GLOBAL_UNIT_ASSIGNED_CONTEXT((#45237,#45239,#45240))
REPRESENTATION_CONTEXT('','3D')
);
#45236=(
GEOMETRIC_REPRESENTATION_CONTEXT(3)
GLOBAL_UNCERTAINTY_ASSIGNED_CONTEXT((#45214))
GLOBAL_UNIT_ASSIGNED_CONTEXT((#45237,#45239,#45240))
REPRESENTATION_CONTEXT('','3D')
);
#45237=(
LENGTH_UNIT()
NAMED_UNIT(*)
SI_UNIT(.MILLI.,.METRE.)
);
#45239=(
NAMED_UNIT(*)
PLANE_ANGLE_UNIT()
SI_UNIT($,.RADIAN.)
);
#45240=(
NAMED_UNIT(*)
SI_UNIT($,.STERADIAN.)
SOLID_ANGLE_UNIT()
);
#45258=SHAPE_DEFINITION_REPRESENTATION(#45279,#45330);
#45279=PRODUCT_DEFINITION_SHAPE('',$,#45352);
#45330=SHAPE_REPRESENTATION('',(#17987),#45232);
#45334=PRODUCT_DEFINITION_CONTEXT('part definition',#45399,'design');
#45352=PRODUCT_DEFINITION('2026-10-25-23-38-19-262',
'09_Plank_Link_Plate',#45373,#45334);
#45373=PRODUCT_DEFINITION_FORMATION('',$,#45418);
#45399=APPLICATION_CONTEXT(
'Core Data for Automotive Mechanical Design Process');
#45400=PRODUCT_CONTEXT('part definition',#45399,'mechanical');
#45418=PRODUCT('2026-10-25-23-38-19-262','09_Plank_Link_Plate',$,(#45400));
#45492=COLOUR_RGB('Off White',0.89,0.88,0.83);
#45493=FILL_AREA_STYLE_COLOUR('',#45492);
#45494=FILL_AREA_STYLE('',(#45493));
#45495=SURFACE_STYLE_FILL_AREA(#45494);
#45496=SURFACE_SIDE_STYLE('',(#45495));
#45497=SURFACE_STYLE_USAGE(.BOTH.,#45496);
#45498=PRESENTATION_STYLE_ASSIGNMENT((#45497));
ENDSEC;
END-ISO-10303-21;
